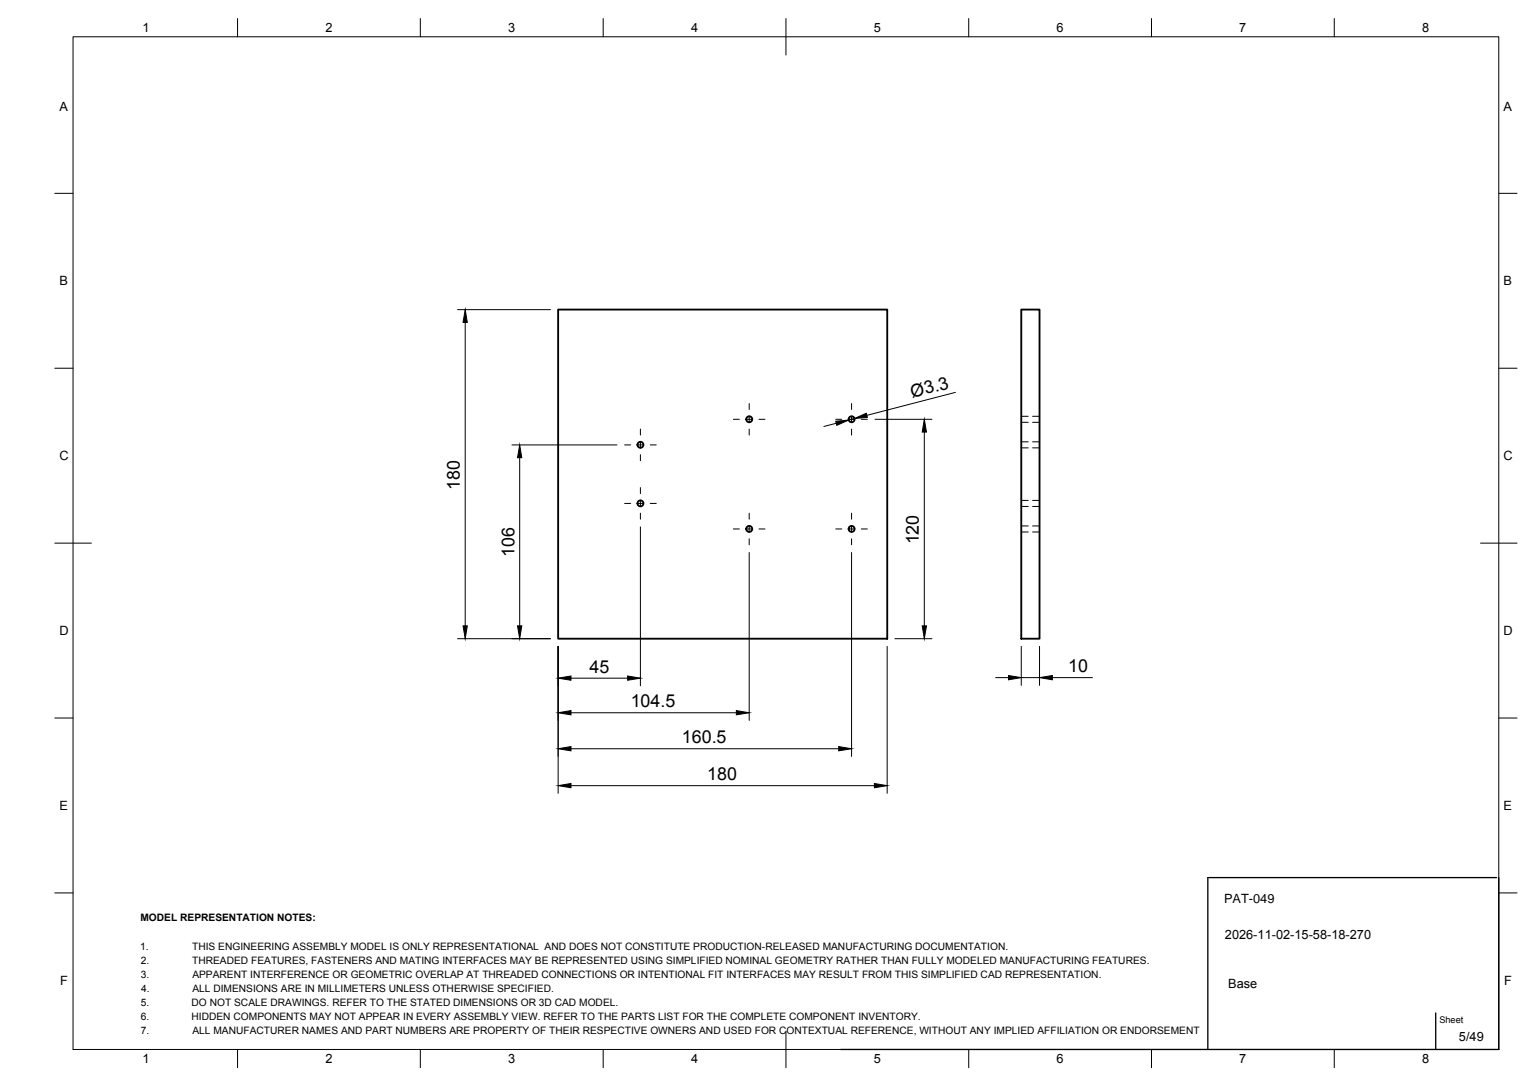
ISO-10303-21;
HEADER;
/* Generated by software containing ST-Developer
 * from STEP Tools, Inc. (www.steptools.com) 
 */

FILE_DESCRIPTION(
/* description */ ('Hand drill press frame (manual)'),
/* implementation_level */ '2;1');

FILE_NAME(
/* name */ 'Base.step',
/* time_stamp */ '2026-10-28T03:25:28-07:00',
/* author */ (''),
/* organization */ (''),
/* preprocessor_version */ 'ST-DEVELOPER v20.2',
/* originating_system */ 'Autodesk Translation Framework v15.17.0.0',
/* authorisation */ '');

FILE_SCHEMA (('AUTOMOTIVE_DESIGN { 1 0 10303 214 3 1 1 }'));
ENDSEC;

DATA;
#10=MECHANICAL_DESIGN_GEOMETRIC_PRESENTATION_REPRESENTATION('',(#619),#33299);
#529=SHAPE_REPRESENTATION_RELATIONSHIP('SRR','None',#33488,#574);
#574=ADVANCED_BREP_SHAPE_REPRESENTATION('',(#671),#33250);
#619=STYLED_ITEM('',(#33793),#671);
#671=MANIFOLD_SOLID_BREP('Body1',#12637);
#720=FACE_BOUND('',#2039,.T.);
#721=FACE_BOUND('',#2040,.T.);
#722=FACE_BOUND('',#2041,.T.);
#723=FACE_BOUND('',#2042,.T.);
#724=FACE_BOUND('',#2043,.T.);
#725=FACE_BOUND('',#2044,.T.);
#726=FACE_BOUND('',#2046,.T.);
#727=FACE_BOUND('',#2047,.T.);
#728=FACE_BOUND('',#2048,.T.);
#729=FACE_BOUND('',#2049,.T.);
#730=FACE_BOUND('',#2050,.T.);
#731=FACE_BOUND('',#2051,.T.);
#887=PLANE('',#13209);
#888=PLANE('',#13210);
#889=PLANE('',#13211);
#890=PLANE('',#13212);
#891=PLANE('',#13213);
#892=PLANE('',#13214);
#1339=FACE_OUTER_BOUND('',#2028,.T.);
#1340=FACE_OUTER_BOUND('',#2029,.T.);
#1341=FACE_OUTER_BOUND('',#2030,.T.);
#1342=FACE_OUTER_BOUND('',#2031,.T.);
#1343=FACE_OUTER_BOUND('',#2032,.T.);
#1344=FACE_OUTER_BOUND('',#2033,.T.);
#1345=FACE_OUTER_BOUND('',#2034,.T.);
#1346=FACE_OUTER_BOUND('',#2035,.T.);
#1347=FACE_OUTER_BOUND('',#2036,.T.);
#1348=FACE_OUTER_BOUND('',#2037,.T.);
#1349=FACE_OUTER_BOUND('',#2038,.T.);
#1350=FACE_OUTER_BOUND('',#2045,.T.);
#2028=EDGE_LOOP('',(#8421,#8422,#8423,#8424));
#2029=EDGE_LOOP('',(#8425,#8426,#8427,#8428));
#2030=EDGE_LOOP('',(#8429,#8430,#8431,#8432));
#2031=EDGE_LOOP('',(#8433,#8434,#8435,#8436));
#2032=EDGE_LOOP('',(#8437,#8438,#8439,#8440));
#2033=EDGE_LOOP('',(#8441,#8442,#8443,#8444));
#2034=EDGE_LOOP('',(#8445,#8446,#8447,#8448));
#2035=EDGE_LOOP('',(#8449,#8450,#8451,#8452));
#2036=EDGE_LOOP('',(#8453,#8454,#8455,#8456));
#2037=EDGE_LOOP('',(#8457,#8458,#8459,#8460));
#2038=EDGE_LOOP('',(#8461,#8462,#8463,#8464));
#2039=EDGE_LOOP('',(#8465));
#2040=EDGE_LOOP('',(#8466));
#2041=EDGE_LOOP('',(#8467));
#2042=EDGE_LOOP('',(#8468));
#2043=EDGE_LOOP('',(#8469));
#2044=EDGE_LOOP('',(#8470));
#2045=EDGE_LOOP('',(#8471,#8472,#8473,#8474));
#2046=EDGE_LOOP('',(#8475));
#2047=EDGE_LOOP('',(#8476));
#2048=EDGE_LOOP('',(#8477));
#2049=EDGE_LOOP('',(#8478));
#2050=EDGE_LOOP('',(#8479));
#2051=EDGE_LOOP('',(#8480));
#2884=LINE('',#17897,#4049);
#2885=LINE('',#17903,#4050);
#2886=LINE('',#17909,#4051);
#2887=LINE('',#17915,#4052);
#2888=LINE('',#17921,#4053);
#2889=LINE('',#17927,#4054);
#2890=LINE('',#17932,#4055);
#2891=LINE('',#17934,#4056);
#2892=LINE('',#17936,#4057);
#2893=LINE('',#17937,#4058);
#2894=LINE('',#17940,#4059);
#2895=LINE('',#17942,#4060);
#2896=LINE('',#17943,#4061);
#2897=LINE('',#17946,#4062);
#2898=LINE('',#17948,#4063);
#2899=LINE('',#17949,#4064);
#2900=LINE('',#17951,#4065);
#2901=LINE('',#17952,#4066);
#4049=VECTOR('',#14377,0.165);
#4050=VECTOR('',#14384,0.165);
#4051=VECTOR('',#14391,0.165);
#4052=VECTOR('',#14398,0.165);
#4053=VECTOR('',#14405,0.165);
#4054=VECTOR('',#14412,0.165);
#4055=VECTOR('',#14417,1.);
#4056=VECTOR('',#14418,1.);
#4057=VECTOR('',#14419,1.);
#4058=VECTOR('',#14420,1.);
#4059=VECTOR('',#14423,1.);
#4060=VECTOR('',#14424,1.);
#4061=VECTOR('',#14425,1.);
#4062=VECTOR('',#14428,1.);
#4063=VECTOR('',#14429,1.);
#4064=VECTOR('',#14430,1.);
#4065=VECTOR('',#14433,1.);
#4066=VECTOR('',#14434,1.);
#5214=CIRCLE('',#13192,0.165);
#5215=CIRCLE('',#13193,0.165);
#5216=CIRCLE('',#13195,0.165);
#5217=CIRCLE('',#13196,0.165);
#5218=CIRCLE('',#13198,0.165);
#5219=CIRCLE('',#13199,0.165);
#5220=CIRCLE('',#13201,0.165);
#5221=CIRCLE('',#13202,0.165);
#5222=CIRCLE('',#13204,0.165);
#5223=CIRCLE('',#13205,0.165);
#5224=CIRCLE('',#13207,0.165);
#5225=CIRCLE('',#13208,0.165);
#5613=VERTEX_POINT('',#17894);
#5614=VERTEX_POINT('',#17896);
#5615=VERTEX_POINT('',#17900);
#5616=VERTEX_POINT('',#17902);
#5617=VERTEX_POINT('',#17906);
#5618=VERTEX_POINT('',#17908);
#5619=VERTEX_POINT('',#17912);
#5620=VERTEX_POINT('',#17914);
#5621=VERTEX_POINT('',#17918);
#5622=VERTEX_POINT('',#17920);
#5623=VERTEX_POINT('',#17924);
#5624=VERTEX_POINT('',#17926);
#5625=VERTEX_POINT('',#17930);
#5626=VERTEX_POINT('',#17931);
#5627=VERTEX_POINT('',#17933);
#5628=VERTEX_POINT('',#17935);
#5629=VERTEX_POINT('',#17939);
#5630=VERTEX_POINT('',#17941);
#5631=VERTEX_POINT('',#17945);
#5632=VERTEX_POINT('',#17947);
#6739=EDGE_CURVE('',#5613,#5613,#5214,.T.);
#6740=EDGE_CURVE('',#5613,#5614,#2884,.T.);
#6741=EDGE_CURVE('',#5614,#5614,#5215,.T.);
#6742=EDGE_CURVE('',#5615,#5615,#5216,.T.);
#6743=EDGE_CURVE('',#5615,#5616,#2885,.T.);
#6744=EDGE_CURVE('',#5616,#5616,#5217,.T.);
#6745=EDGE_CURVE('',#5617,#5617,#5218,.T.);
#6746=EDGE_CURVE('',#5617,#5618,#2886,.T.);
#6747=EDGE_CURVE('',#5618,#5618,#5219,.T.);
#6748=EDGE_CURVE('',#5619,#5619,#5220,.T.);
#6749=EDGE_CURVE('',#5619,#5620,#2887,.T.);
#6750=EDGE_CURVE('',#5620,#5620,#5221,.T.);
#6751=EDGE_CURVE('',#5621,#5621,#5222,.T.);
#6752=EDGE_CURVE('',#5621,#5622,#2888,.T.);
#6753=EDGE_CURVE('',#5622,#5622,#5223,.T.);
#6754=EDGE_CURVE('',#5623,#5623,#5224,.T.);
#6755=EDGE_CURVE('',#5623,#5624,#2889,.T.);
#6756=EDGE_CURVE('',#5624,#5624,#5225,.T.);
#6757=EDGE_CURVE('',#5625,#5626,#2890,.T.);
#6758=EDGE_CURVE('',#5626,#5627,#2891,.T.);
#6759=EDGE_CURVE('',#5628,#5627,#2892,.T.);
#6760=EDGE_CURVE('',#5625,#5628,#2893,.T.);
#6761=EDGE_CURVE('',#5629,#5625,#2894,.T.);
#6762=EDGE_CURVE('',#5630,#5628,#2895,.T.);
#6763=EDGE_CURVE('',#5629,#5630,#2896,.T.);
#6764=EDGE_CURVE('',#5631,#5629,#2897,.T.);
#6765=EDGE_CURVE('',#5632,#5630,#2898,.T.);
#6766=EDGE_CURVE('',#5631,#5632,#2899,.T.);
#6767=EDGE_CURVE('',#5626,#5631,#2900,.T.);
#6768=EDGE_CURVE('',#5627,#5632,#2901,.T.);
#8421=ORIENTED_EDGE('',*,*,#6739,.F.);
#8422=ORIENTED_EDGE('',*,*,#6740,.T.);
#8423=ORIENTED_EDGE('',*,*,#6741,.F.);
#8424=ORIENTED_EDGE('',*,*,#6740,.F.);
#8425=ORIENTED_EDGE('',*,*,#6742,.F.);
#8426=ORIENTED_EDGE('',*,*,#6743,.T.);
#8427=ORIENTED_EDGE('',*,*,#6744,.F.);
#8428=ORIENTED_EDGE('',*,*,#6743,.F.);
#8429=ORIENTED_EDGE('',*,*,#6745,.F.);
#8430=ORIENTED_EDGE('',*,*,#6746,.T.);
#8431=ORIENTED_EDGE('',*,*,#6747,.F.);
#8432=ORIENTED_EDGE('',*,*,#6746,.F.);
#8433=ORIENTED_EDGE('',*,*,#6748,.F.);
#8434=ORIENTED_EDGE('',*,*,#6749,.T.);
#8435=ORIENTED_EDGE('',*,*,#6750,.F.);
#8436=ORIENTED_EDGE('',*,*,#6749,.F.);
#8437=ORIENTED_EDGE('',*,*,#6751,.F.);
#8438=ORIENTED_EDGE('',*,*,#6752,.T.);
#8439=ORIENTED_EDGE('',*,*,#6753,.F.);
#8440=ORIENTED_EDGE('',*,*,#6752,.F.);
#8441=ORIENTED_EDGE('',*,*,#6754,.F.);
#8442=ORIENTED_EDGE('',*,*,#6755,.T.);
#8443=ORIENTED_EDGE('',*,*,#6756,.F.);
#8444=ORIENTED_EDGE('',*,*,#6755,.F.);
#8445=ORIENTED_EDGE('',*,*,#6757,.T.);
#8446=ORIENTED_EDGE('',*,*,#6758,.T.);
#8447=ORIENTED_EDGE('',*,*,#6759,.F.);
#8448=ORIENTED_EDGE('',*,*,#6760,.F.);
#8449=ORIENTED_EDGE('',*,*,#6761,.T.);
#8450=ORIENTED_EDGE('',*,*,#6760,.T.);
#8451=ORIENTED_EDGE('',*,*,#6762,.F.);
#8452=ORIENTED_EDGE('',*,*,#6763,.F.);
#8453=ORIENTED_EDGE('',*,*,#6764,.T.);
#8454=ORIENTED_EDGE('',*,*,#6763,.T.);
#8455=ORIENTED_EDGE('',*,*,#6765,.F.);
#8456=ORIENTED_EDGE('',*,*,#6766,.F.);
#8457=ORIENTED_EDGE('',*,*,#6767,.T.);
#8458=ORIENTED_EDGE('',*,*,#6766,.T.);
#8459=ORIENTED_EDGE('',*,*,#6768,.F.);
#8460=ORIENTED_EDGE('',*,*,#6758,.F.);
#8461=ORIENTED_EDGE('',*,*,#6768,.T.);
#8462=ORIENTED_EDGE('',*,*,#6765,.T.);
#8463=ORIENTED_EDGE('',*,*,#6762,.T.);
#8464=ORIENTED_EDGE('',*,*,#6759,.T.);
#8465=ORIENTED_EDGE('',*,*,#6741,.T.);
#8466=ORIENTED_EDGE('',*,*,#6744,.T.);
#8467=ORIENTED_EDGE('',*,*,#6747,.T.);
#8468=ORIENTED_EDGE('',*,*,#6750,.T.);
#8469=ORIENTED_EDGE('',*,*,#6753,.T.);
#8470=ORIENTED_EDGE('',*,*,#6756,.T.);
#8471=ORIENTED_EDGE('',*,*,#6767,.F.);
#8472=ORIENTED_EDGE('',*,*,#6757,.F.);
#8473=ORIENTED_EDGE('',*,*,#6761,.F.);
#8474=ORIENTED_EDGE('',*,*,#6764,.F.);
#8475=ORIENTED_EDGE('',*,*,#6739,.T.);
#8476=ORIENTED_EDGE('',*,*,#6742,.T.);
#8477=ORIENTED_EDGE('',*,*,#6745,.T.);
#8478=ORIENTED_EDGE('',*,*,#6748,.T.);
#8479=ORIENTED_EDGE('',*,*,#6751,.T.);
#8480=ORIENTED_EDGE('',*,*,#6754,.T.);
#11785=CYLINDRICAL_SURFACE('',#13191,0.165);
#11786=CYLINDRICAL_SURFACE('',#13194,0.165);
#11787=CYLINDRICAL_SURFACE('',#13197,0.165);
#11788=CYLINDRICAL_SURFACE('',#13200,0.165);
#11789=CYLINDRICAL_SURFACE('',#13203,0.165);
#11790=CYLINDRICAL_SURFACE('',#13206,0.165);
#11948=ADVANCED_FACE('',(#1339),#11785,.F.);
#11949=ADVANCED_FACE('',(#1340),#11786,.F.);
#11950=ADVANCED_FACE('',(#1341),#11787,.F.);
#11951=ADVANCED_FACE('',(#1342),#11788,.F.);
#11952=ADVANCED_FACE('',(#1343),#11789,.F.);
#11953=ADVANCED_FACE('',(#1344),#11790,.F.);
#11954=ADVANCED_FACE('',(#1345),#887,.T.);
#11955=ADVANCED_FACE('',(#1346),#888,.T.);
#11956=ADVANCED_FACE('',(#1347),#889,.T.);
#11957=ADVANCED_FACE('',(#1348),#890,.T.);
#11958=ADVANCED_FACE('',(#1349,#720,#721,#722,#723,#724,#725),#891,.T.);
#11959=ADVANCED_FACE('',(#1350,#726,#727,#728,#729,#730,#731),#892,.F.);
#12637=CLOSED_SHELL('',(#11948,#11949,#11950,#11951,#11952,#11953,#11954,
#11955,#11956,#11957,#11958,#11959));
#13190=AXIS2_PLACEMENT_3D('',#17892,#14371,#14372);
#13191=AXIS2_PLACEMENT_3D('',#17893,#14373,#14374);
#13192=AXIS2_PLACEMENT_3D('',#17895,#14375,#14376);
#13193=AXIS2_PLACEMENT_3D('',#17898,#14378,#14379);
#13194=AXIS2_PLACEMENT_3D('',#17899,#14380,#14381);
#13195=AXIS2_PLACEMENT_3D('',#17901,#14382,#14383);
#13196=AXIS2_PLACEMENT_3D('',#17904,#14385,#14386);
#13197=AXIS2_PLACEMENT_3D('',#17905,#14387,#14388);
#13198=AXIS2_PLACEMENT_3D('',#17907,#14389,#14390);
#13199=AXIS2_PLACEMENT_3D('',#17910,#14392,#14393);
#13200=AXIS2_PLACEMENT_3D('',#17911,#14394,#14395);
#13201=AXIS2_PLACEMENT_3D('',#17913,#14396,#14397);
#13202=AXIS2_PLACEMENT_3D('',#17916,#14399,#14400);
#13203=AXIS2_PLACEMENT_3D('',#17917,#14401,#14402);
#13204=AXIS2_PLACEMENT_3D('',#17919,#14403,#14404);
#13205=AXIS2_PLACEMENT_3D('',#17922,#14406,#14407);
#13206=AXIS2_PLACEMENT_3D('',#17923,#14408,#14409);
#13207=AXIS2_PLACEMENT_3D('',#17925,#14410,#14411);
#13208=AXIS2_PLACEMENT_3D('',#17928,#14413,#14414);
#13209=AXIS2_PLACEMENT_3D('',#17929,#14415,#14416);
#13210=AXIS2_PLACEMENT_3D('',#17938,#14421,#14422);
#13211=AXIS2_PLACEMENT_3D('',#17944,#14426,#14427);
#13212=AXIS2_PLACEMENT_3D('',#17950,#14431,#14432);
#13213=AXIS2_PLACEMENT_3D('',#17953,#14435,#14436);
#13214=AXIS2_PLACEMENT_3D('',#17954,#14437,#14438);
#14371=DIRECTION('axis',(0.,0.,1.));
#14372=DIRECTION('refdir',(1.,0.,0.));
#14373=DIRECTION('center_axis',(0.,0.,1.));
#14374=DIRECTION('ref_axis',(1.,0.,0.));
#14375=DIRECTION('center_axis',(0.,0.,1.));
#14376=DIRECTION('ref_axis',(1.,0.,0.));
#14377=DIRECTION('',(0.,0.,1.));
#14378=DIRECTION('center_axis',(0.,0.,-1.));
#14379=DIRECTION('ref_axis',(1.,0.,0.));
#14380=DIRECTION('center_axis',(0.,0.,1.));
#14381=DIRECTION('ref_axis',(1.,0.,0.));
#14382=DIRECTION('center_axis',(0.,0.,1.));
#14383=DIRECTION('ref_axis',(1.,0.,0.));
#14384=DIRECTION('',(0.,0.,1.));
#14385=DIRECTION('center_axis',(0.,0.,-1.));
#14386=DIRECTION('ref_axis',(1.,0.,0.));
#14387=DIRECTION('center_axis',(0.,0.,1.));
#14388=DIRECTION('ref_axis',(1.,0.,0.));
#14389=DIRECTION('center_axis',(0.,0.,1.));
#14390=DIRECTION('ref_axis',(1.,0.,0.));
#14391=DIRECTION('',(0.,0.,1.));
#14392=DIRECTION('center_axis',(0.,0.,-1.));
#14393=DIRECTION('ref_axis',(1.,0.,0.));
#14394=DIRECTION('center_axis',(0.,0.,1.));
#14395=DIRECTION('ref_axis',(1.,0.,0.));
#14396=DIRECTION('center_axis',(0.,0.,1.));
#14397=DIRECTION('ref_axis',(1.,0.,0.));
#14398=DIRECTION('',(0.,0.,1.));
#14399=DIRECTION('center_axis',(0.,0.,-1.));
#14400=DIRECTION('ref_axis',(1.,0.,0.));
#14401=DIRECTION('center_axis',(0.,0.,1.));
#14402=DIRECTION('ref_axis',(1.,0.,0.));
#14403=DIRECTION('center_axis',(0.,0.,1.));
#14404=DIRECTION('ref_axis',(1.,0.,0.));
#14405=DIRECTION('',(0.,0.,1.));
#14406=DIRECTION('center_axis',(0.,0.,-1.));
#14407=DIRECTION('ref_axis',(1.,0.,0.));
#14408=DIRECTION('center_axis',(0.,0.,1.));
#14409=DIRECTION('ref_axis',(1.,0.,0.));
#14410=DIRECTION('center_axis',(0.,0.,1.));
#14411=DIRECTION('ref_axis',(1.,0.,0.));
#14412=DIRECTION('',(0.,0.,1.));
#14413=DIRECTION('center_axis',(0.,0.,-1.));
#14414=DIRECTION('ref_axis',(1.,0.,0.));
#14415=DIRECTION('center_axis',(0.,1.,0.));
#14416=DIRECTION('ref_axis',(-1.,0.,0.));
#14417=DIRECTION('',(-1.,0.,0.));
#14418=DIRECTION('',(0.,0.,1.));
#14419=DIRECTION('',(-1.,0.,0.));
#14420=DIRECTION('',(0.,0.,1.));
#14421=DIRECTION('center_axis',(1.,0.,0.));
#14422=DIRECTION('ref_axis',(0.,1.,0.));
#14423=DIRECTION('',(0.,1.,0.));
#14424=DIRECTION('',(0.,1.,0.));
#14425=DIRECTION('',(0.,0.,1.));
#14426=DIRECTION('center_axis',(0.,-1.,0.));
#14427=DIRECTION('ref_axis',(1.,0.,0.));
#14428=DIRECTION('',(1.,0.,0.));
#14429=DIRECTION('',(1.,0.,0.));
#14430=DIRECTION('',(0.,0.,1.));
#14431=DIRECTION('center_axis',(-1.,0.,0.));
#14432=DIRECTION('ref_axis',(0.,-1.,0.));
#14433=DIRECTION('',(0.,-1.,0.));
#14434=DIRECTION('',(0.,-1.,0.));
#14435=DIRECTION('center_axis',(0.,0.,1.));
#14436=DIRECTION('ref_axis',(1.,0.,0.));
#14437=DIRECTION('center_axis',(0.,0.,1.));
#14438=DIRECTION('ref_axis',(1.,0.,0.));
#17892=CARTESIAN_POINT('',(0.,0.,0.));
#17893=CARTESIAN_POINT('Origin',(-6.05,3.,-0.1));
#17894=CARTESIAN_POINT('',(-6.215,3.,0.));
#17895=CARTESIAN_POINT('Origin',(-6.05,3.,0.));
#17896=CARTESIAN_POINT('',(-6.215,3.,1.));
#17897=CARTESIAN_POINT('',(-6.215,3.,-0.1));
#17898=CARTESIAN_POINT('Origin',(-6.05,3.,1.));
#17899=CARTESIAN_POINT('Origin',(-0.45,3.,-0.1));
#17900=CARTESIAN_POINT('',(-0.615,3.,0.));
#17901=CARTESIAN_POINT('Origin',(-0.45,3.,0.));
#17902=CARTESIAN_POINT('',(-0.615,3.,1.));
#17903=CARTESIAN_POINT('',(-0.615,3.,-0.1));
#17904=CARTESIAN_POINT('Origin',(-0.45,3.,1.));
#17905=CARTESIAN_POINT('Origin',(-6.05,-3.,-0.1));
#17906=CARTESIAN_POINT('',(-6.215,-3.,0.));
#17907=CARTESIAN_POINT('Origin',(-6.05,-3.,0.));
#17908=CARTESIAN_POINT('',(-6.215,-3.,1.));
#17909=CARTESIAN_POINT('',(-6.215,-3.,-0.1));
#17910=CARTESIAN_POINT('Origin',(-6.05,-3.,1.));
#17911=CARTESIAN_POINT('Origin',(-0.45,-3.,-0.1));
#17912=CARTESIAN_POINT('',(-0.615,-3.,0.));
#17913=CARTESIAN_POINT('Origin',(-0.45,-3.,0.));
#17914=CARTESIAN_POINT('',(-0.615,-3.,1.));
#17915=CARTESIAN_POINT('',(-0.615,-3.,-0.1));
#17916=CARTESIAN_POINT('Origin',(-0.45,-3.,1.));
#17917=CARTESIAN_POINT('Origin',(5.5,-1.6,-0.1));
#17918=CARTESIAN_POINT('',(5.335,-1.6,0.));
#17919=CARTESIAN_POINT('Origin',(5.5,-1.6,0.));
#17920=CARTESIAN_POINT('',(5.335,-1.6,1.));
#17921=CARTESIAN_POINT('',(5.335,-1.6,-0.1));
#17922=CARTESIAN_POINT('Origin',(5.5,-1.6,1.));
#17923=CARTESIAN_POINT('Origin',(5.5,1.6,-0.1));
#17924=CARTESIAN_POINT('',(5.335,1.6,0.));
#17925=CARTESIAN_POINT('Origin',(5.5,1.6,0.));
#17926=CARTESIAN_POINT('',(5.335,1.6,1.));
#17927=CARTESIAN_POINT('',(5.335,1.6,-0.1));
#17928=CARTESIAN_POINT('Origin',(5.5,1.6,1.));
#17929=CARTESIAN_POINT('Origin',(10.,9.,0.));
#17930=CARTESIAN_POINT('',(10.,9.,0.));
#17931=CARTESIAN_POINT('',(-8.,9.,0.));
#17932=CARTESIAN_POINT('',(10.,9.,0.));
#17933=CARTESIAN_POINT('',(-8.,9.,1.));
#17934=CARTESIAN_POINT('',(-8.,9.,0.));
#17935=CARTESIAN_POINT('',(10.,9.,1.));
#17936=CARTESIAN_POINT('',(10.,9.,1.));
#17937=CARTESIAN_POINT('',(10.,9.,0.));
#17938=CARTESIAN_POINT('Origin',(10.,-9.,0.));
#17939=CARTESIAN_POINT('',(10.,-9.,0.));
#17940=CARTESIAN_POINT('',(10.,-9.,0.));
#17941=CARTESIAN_POINT('',(10.,-9.,1.));
#17942=CARTESIAN_POINT('',(10.,-9.,1.));
#17943=CARTESIAN_POINT('',(10.,-9.,0.));
#17944=CARTESIAN_POINT('Origin',(-8.,-9.,0.));
#17945=CARTESIAN_POINT('',(-8.,-9.,0.));
#17946=CARTESIAN_POINT('',(-8.,-9.,0.));
#17947=CARTESIAN_POINT('',(-8.,-9.,1.));
#17948=CARTESIAN_POINT('',(-8.,-9.,1.));
#17949=CARTESIAN_POINT('',(-8.,-9.,0.));
#17950=CARTESIAN_POINT('Origin',(-8.,9.,0.));
#17951=CARTESIAN_POINT('',(-8.,9.,0.));
#17952=CARTESIAN_POINT('',(-8.,9.,1.));
#17953=CARTESIAN_POINT('Origin',(1.,0.,1.));
#17954=CARTESIAN_POINT('Origin',(1.,0.,0.));
#33198=UNCERTAINTY_MEASURE_WITH_UNIT(LENGTH_MEASURE(0.001),#33300,
'DISTANCE_ACCURACY_VALUE',
'Maximum model space distance between geometric entities at asserted c
onnectivities');
#33247=UNCERTAINTY_MEASURE_WITH_UNIT(LENGTH_MEASURE(0.001),#33300,
'DISTANCE_ACCURACY_VALUE',
'Maximum model space distance between geometric entities at asserted c
onnectivities');
#33250=(
GEOMETRIC_REPRESENTATION_CONTEXT(3)
GLOBAL_UNCERTAINTY_ASSIGNED_CONTEXT((#33198))
GLOBAL_UNIT_ASSIGNED_CONTEXT((#33300,#33302,#33303))
REPRESENTATION_CONTEXT('','3D')
);
#33299=(
GEOMETRIC_REPRESENTATION_CONTEXT(3)
GLOBAL_UNCERTAINTY_ASSIGNED_CONTEXT((#33247))
GLOBAL_UNIT_ASSIGNED_CONTEXT((#33300,#33302,#33303))
REPRESENTATION_CONTEXT('','3D')
);
#33300=(
LENGTH_UNIT()
NAMED_UNIT(*)
SI_UNIT(.CENTI.,.METRE.)
);
#33302=(
NAMED_UNIT(*)
PLANE_ANGLE_UNIT()
SI_UNIT($,.RADIAN.)
);
#33303=(
NAMED_UNIT(*)
SI_UNIT($,.STERADIAN.)
SOLID_ANGLE_UNIT()
);
#33306=SHAPE_DEFINITION_REPRESENTATION(#33357,#33488);
#33357=PRODUCT_DEFINITION_SHAPE('',$,#33540);
#33488=SHAPE_REPRESENTATION('',(#13190),#33250);
#33537=PRODUCT_DEFINITION_CONTEXT('part definition',#33692,'design');
#33540=PRODUCT_DEFINITION('Base','Base',#33591,#33537);
#33591=PRODUCT_DEFINITION_FORMATION('',$,#33696);
#33692=APPLICATION_CONTEXT(
'Core Data for Automotive Mechanical Design Process');
#33693=PRODUCT_CONTEXT('part definition',#33692,'mechanical');
#33696=PRODUCT('Base','Base','Base',(#33693));
#33787=COLOUR_RGB('Dark Blue',0.08,0.2,0.34);
#33788=FILL_AREA_STYLE_COLOUR('',#33787);
#33789=FILL_AREA_STYLE('',(#33788));
#33790=SURFACE_STYLE_FILL_AREA(#33789);
#33791=SURFACE_SIDE_STYLE('',(#33790));
#33792=SURFACE_STYLE_USAGE(.BOTH.,#33791);
#33793=PRESENTATION_STYLE_ASSIGNMENT((#33792));
ENDSEC;
END-ISO-10303-21;
